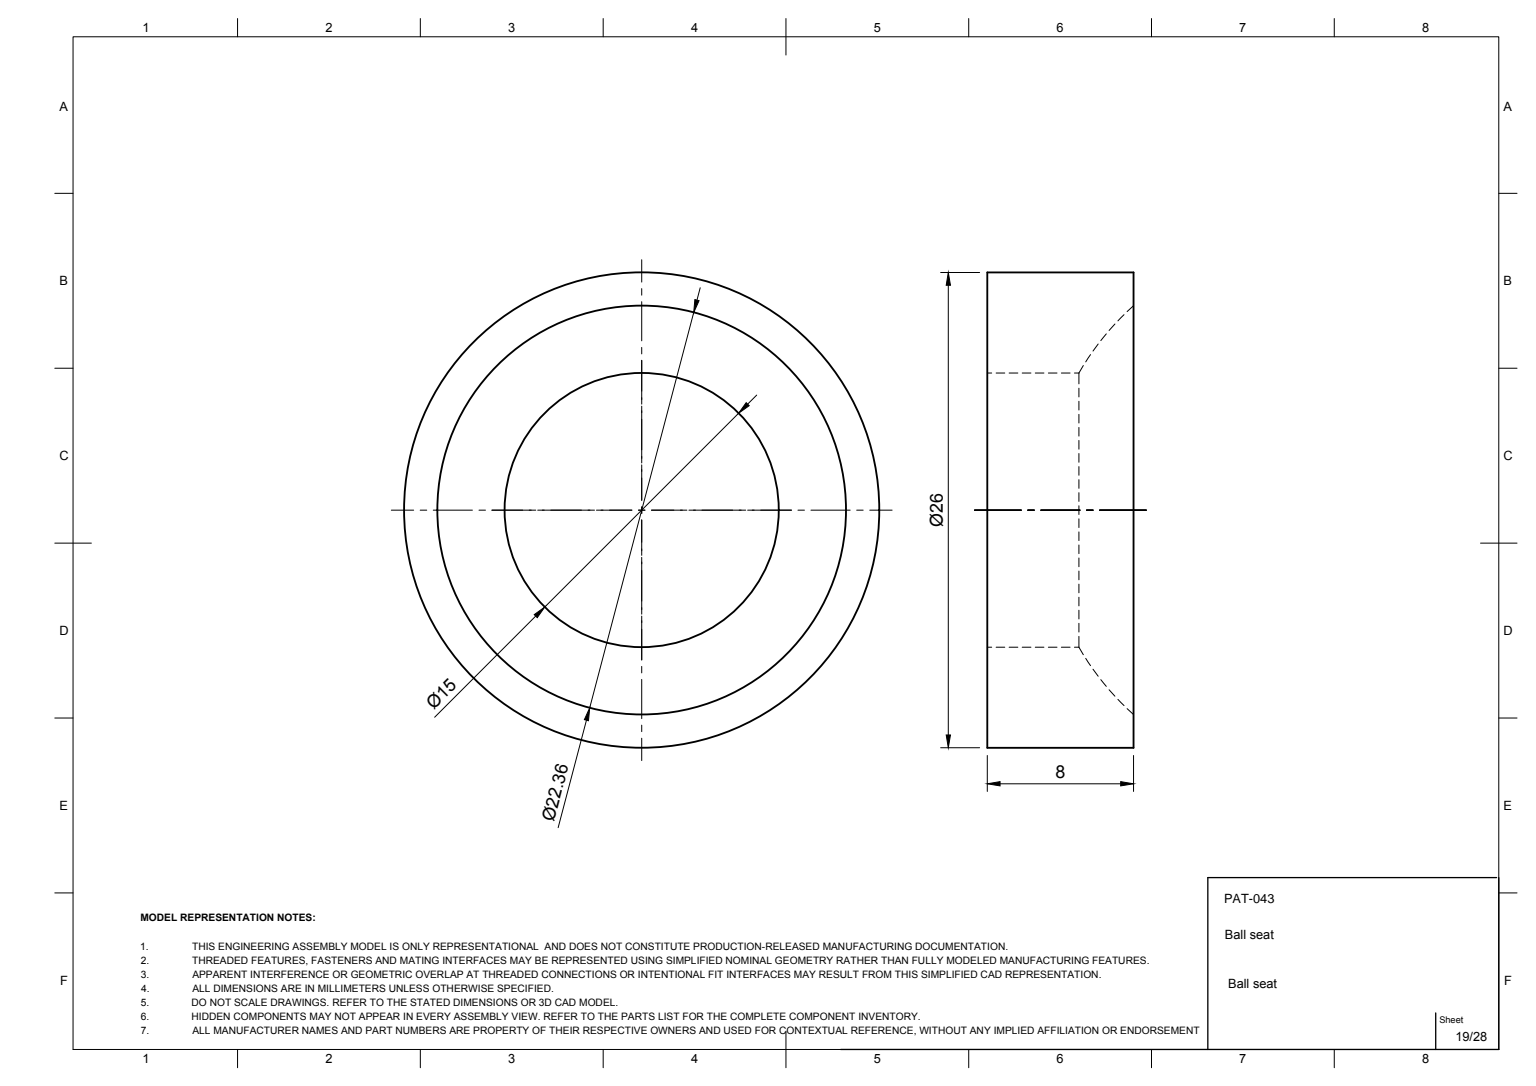
ISO-10303-21;
HEADER;
/* Generated by software containing ST-Developer
 * from STEP Tools, Inc. (www.steptools.com) 
 */

FILE_DESCRIPTION(
/* description */ ('Four-valve pipe header'),
/* implementation_level */ '2;1');

FILE_NAME(
/* name */ 'Ball seat.step',
/* time_stamp */ '2026-10-29T16:56:19-07:00',
/* author */ (''),
/* organization */ (''),
/* preprocessor_version */ 'ST-DEVELOPER v20.2',
/* originating_system */ 'Autodesk Translation Framework v15.17.0.0',
/* authorisation */ '');

FILE_SCHEMA (('AUTOMOTIVE_DESIGN { 1 0 10303 214 3 1 1 }'));
ENDSEC;

DATA;
#10=MECHANICAL_DESIGN_GEOMETRIC_PRESENTATION_REPRESENTATION('',(#345),#10119);
#244=SPHERICAL_SURFACE('',#6280,1.5);
#293=SHAPE_REPRESENTATION_RELATIONSHIP('SRR','None',#10255,#319);
#319=ADVANCED_BREP_SHAPE_REPRESENTATION('',(#371),#10104);
#345=STYLED_ITEM('',(#10456),#371);
#371=MANIFOLD_SOLID_BREP('Body1',#5591);
#510=FACE_BOUND('',#1353,.T.);
#511=FACE_BOUND('',#1357,.T.);
#512=FACE_BOUND('',#1359,.T.);
#644=PLANE('',#6288);
#645=PLANE('',#6289);
#936=FACE_OUTER_BOUND('',#1352,.T.);
#937=FACE_OUTER_BOUND('',#1354,.T.);
#938=FACE_OUTER_BOUND('',#1355,.T.);
#939=FACE_OUTER_BOUND('',#1356,.T.);
#940=FACE_OUTER_BOUND('',#1358,.T.);
#1352=EDGE_LOOP('',(#4589));
#1353=EDGE_LOOP('',(#4590));
#1354=EDGE_LOOP('',(#4591,#4592,#4593,#4594));
#1355=EDGE_LOOP('',(#4595,#4596,#4597,#4598));
#1356=EDGE_LOOP('',(#4599));
#1357=EDGE_LOOP('',(#4600));
#1358=EDGE_LOOP('',(#4601));
#1359=EDGE_LOOP('',(#4602));
#1746=LINE('',#9368,#2164);
#1747=LINE('',#9374,#2165);
#2164=VECTOR('',#7573,0.75);
#2165=VECTOR('',#7580,1.3);
#2504=CIRCLE('',#6281,1.11803398874989);
#2505=CIRCLE('',#6282,0.75);
#2506=CIRCLE('',#6284,0.75);
#2507=CIRCLE('',#6286,1.3);
#2508=CIRCLE('',#6287,1.3);
#2857=VERTEX_POINT('',#9362);
#2858=VERTEX_POINT('',#9364);
#2859=VERTEX_POINT('',#9367);
#2860=VERTEX_POINT('',#9371);
#2861=VERTEX_POINT('',#9373);
#3461=EDGE_CURVE('',#2857,#2857,#2504,.T.);
#3462=EDGE_CURVE('',#2858,#2858,#2505,.T.);
#3463=EDGE_CURVE('',#2858,#2859,#1746,.T.);
#3464=EDGE_CURVE('',#2859,#2859,#2506,.T.);
#3465=EDGE_CURVE('',#2860,#2860,#2507,.T.);
#3466=EDGE_CURVE('',#2860,#2861,#1747,.T.);
#3467=EDGE_CURVE('',#2861,#2861,#2508,.T.);
#4589=ORIENTED_EDGE('',*,*,#3461,.F.);
#4590=ORIENTED_EDGE('',*,*,#3462,.F.);
#4591=ORIENTED_EDGE('',*,*,#3462,.T.);
#4592=ORIENTED_EDGE('',*,*,#3463,.T.);
#4593=ORIENTED_EDGE('',*,*,#3464,.T.);
#4594=ORIENTED_EDGE('',*,*,#3463,.F.);
#4595=ORIENTED_EDGE('',*,*,#3465,.F.);
#4596=ORIENTED_EDGE('',*,*,#3466,.T.);
#4597=ORIENTED_EDGE('',*,*,#3467,.T.);
#4598=ORIENTED_EDGE('',*,*,#3466,.F.);
#4599=ORIENTED_EDGE('',*,*,#3465,.T.);
#4600=ORIENTED_EDGE('',*,*,#3461,.T.);
#4601=ORIENTED_EDGE('',*,*,#3467,.F.);
#4602=ORIENTED_EDGE('',*,*,#3464,.F.);
#5224=CYLINDRICAL_SURFACE('',#6283,0.75);
#5225=CYLINDRICAL_SURFACE('',#6285,1.3);
#5436=ADVANCED_FACE('',(#936,#510),#244,.F.);
#5437=ADVANCED_FACE('',(#937),#5224,.F.);
#5438=ADVANCED_FACE('',(#938),#5225,.T.);
#5439=ADVANCED_FACE('',(#939,#511),#644,.T.);
#5440=ADVANCED_FACE('',(#940,#512),#645,.F.);
#5591=CLOSED_SHELL('',(#5436,#5437,#5438,#5439,#5440));
#6279=AXIS2_PLACEMENT_3D('',#9360,#7563,#7564);
#6280=AXIS2_PLACEMENT_3D('',#9361,#7565,#7566);
#6281=AXIS2_PLACEMENT_3D('',#9363,#7567,#7568);
#6282=AXIS2_PLACEMENT_3D('',#9365,#7569,#7570);
#6283=AXIS2_PLACEMENT_3D('',#9366,#7571,#7572);
#6284=AXIS2_PLACEMENT_3D('',#9369,#7574,#7575);
#6285=AXIS2_PLACEMENT_3D('',#9370,#7576,#7577);
#6286=AXIS2_PLACEMENT_3D('',#9372,#7578,#7579);
#6287=AXIS2_PLACEMENT_3D('',#9375,#7581,#7582);
#6288=AXIS2_PLACEMENT_3D('',#9376,#7583,#7584);
#6289=AXIS2_PLACEMENT_3D('',#9377,#7585,#7586);
#7563=DIRECTION('axis',(0.,0.,1.));
#7564=DIRECTION('refdir',(1.,0.,0.));
#7565=DIRECTION('center_axis',(6.12323399573677E-17,0.,1.));
#7566=DIRECTION('ref_axis',(1.,0.,0.));
#7567=DIRECTION('center_axis',(0.,-1.,0.));
#7568=DIRECTION('ref_axis',(0.,0.,-1.));
#7569=DIRECTION('center_axis',(0.,1.,0.));
#7570=DIRECTION('ref_axis',(1.,0.,0.));
#7571=DIRECTION('center_axis',(0.,1.,0.));
#7572=DIRECTION('ref_axis',(1.,0.,0.));
#7573=DIRECTION('',(0.,-1.,0.));
#7574=DIRECTION('center_axis',(0.,-1.,0.));
#7575=DIRECTION('ref_axis',(1.,0.,0.));
#7576=DIRECTION('center_axis',(0.,1.,0.));
#7577=DIRECTION('ref_axis',(1.,0.,0.));
#7578=DIRECTION('center_axis',(0.,1.,0.));
#7579=DIRECTION('ref_axis',(1.,0.,0.));
#7580=DIRECTION('',(0.,-1.,0.));
#7581=DIRECTION('center_axis',(0.,1.,0.));
#7582=DIRECTION('ref_axis',(1.,0.,0.));
#7583=DIRECTION('center_axis',(0.,1.,0.));
#7584=DIRECTION('ref_axis',(1.,0.,0.));
#7585=DIRECTION('center_axis',(0.,1.,0.));
#7586=DIRECTION('ref_axis',(1.,0.,0.));
#9360=CARTESIAN_POINT('',(0.,0.,0.));
#9361=CARTESIAN_POINT('Origin',(0.,0.,5.));
#9362=CARTESIAN_POINT('',(-1.36919674566051E-16,-1.,6.11803398874989));
#9363=CARTESIAN_POINT('Origin',(0.,-1.,5.));
#9364=CARTESIAN_POINT('',(-0.75,-1.29903810567666,5.));
#9365=CARTESIAN_POINT('Origin',(0.,-1.29903810567666,5.));
#9366=CARTESIAN_POINT('Origin',(0.,-1.8,5.));
#9367=CARTESIAN_POINT('',(-0.75,-1.8,5.));
#9368=CARTESIAN_POINT('',(-0.75,-1.8,5.));
#9369=CARTESIAN_POINT('Origin',(0.,-1.8,5.));
#9370=CARTESIAN_POINT('Origin',(0.,-1.8,5.));
#9371=CARTESIAN_POINT('',(-1.3,-1.,5.));
#9372=CARTESIAN_POINT('Origin',(0.,-1.,5.));
#9373=CARTESIAN_POINT('',(-1.3,-1.8,5.));
#9374=CARTESIAN_POINT('',(-1.3,-1.8,5.));
#9375=CARTESIAN_POINT('Origin',(0.,-1.8,5.));
#9376=CARTESIAN_POINT('Origin',(0.,-1.,5.));
#9377=CARTESIAN_POINT('Origin',(0.,-1.8,5.));
#10073=UNCERTAINTY_MEASURE_WITH_UNIT(LENGTH_MEASURE(0.001),#10120,
'DISTANCE_ACCURACY_VALUE',
'Maximum model space distance between geometric entities at asserted c
onnectivities');
#10088=UNCERTAINTY_MEASURE_WITH_UNIT(LENGTH_MEASURE(0.001),#10120,
'DISTANCE_ACCURACY_VALUE',
'Maximum model space distance between geometric entities at asserted c
onnectivities');
#10104=(
GEOMETRIC_REPRESENTATION_CONTEXT(3)
GLOBAL_UNCERTAINTY_ASSIGNED_CONTEXT((#10073))
GLOBAL_UNIT_ASSIGNED_CONTEXT((#10120,#10122,#10123))
REPRESENTATION_CONTEXT('','3D')
);
#10119=(
GEOMETRIC_REPRESENTATION_CONTEXT(3)
GLOBAL_UNCERTAINTY_ASSIGNED_CONTEXT((#10088))
GLOBAL_UNIT_ASSIGNED_CONTEXT((#10120,#10122,#10123))
REPRESENTATION_CONTEXT('','3D')
);
#10120=(
LENGTH_UNIT()
NAMED_UNIT(*)
SI_UNIT(.CENTI.,.METRE.)
);
#10122=(
NAMED_UNIT(*)
PLANE_ANGLE_UNIT()
SI_UNIT($,.RADIAN.)
);
#10123=(
NAMED_UNIT(*)
SI_UNIT($,.STERADIAN.)
SOLID_ANGLE_UNIT()
);
#10139=SHAPE_DEFINITION_REPRESENTATION(#10169,#10255);
#10169=PRODUCT_DEFINITION_SHAPE('',$,#10286);
#10255=SHAPE_REPRESENTATION('',(#6279),#10104);
#10270=PRODUCT_DEFINITION_CONTEXT('part definition',#10362,'design');
#10286=PRODUCT_DEFINITION('Ball seat','Ball seat',#10316,#10270);
#10316=PRODUCT_DEFINITION_FORMATION('',$,#10379);
#10362=APPLICATION_CONTEXT(
'Core Data for Automotive Mechanical Design Process');
#10363=PRODUCT_CONTEXT('part definition',#10362,'mechanical');
#10379=PRODUCT('Ball seat','Ball seat','Ball seat',(#10363));
#10450=COLOUR_RGB('Light Blue',0.38,0.62,0.78);
#10451=FILL_AREA_STYLE_COLOUR('',#10450);
#10452=FILL_AREA_STYLE('',(#10451));
#10453=SURFACE_STYLE_FILL_AREA(#10452);
#10454=SURFACE_SIDE_STYLE('',(#10453));
#10455=SURFACE_STYLE_USAGE(.BOTH.,#10454);
#10456=PRESENTATION_STYLE_ASSIGNMENT((#10455));
ENDSEC;
END-ISO-10303-21;
